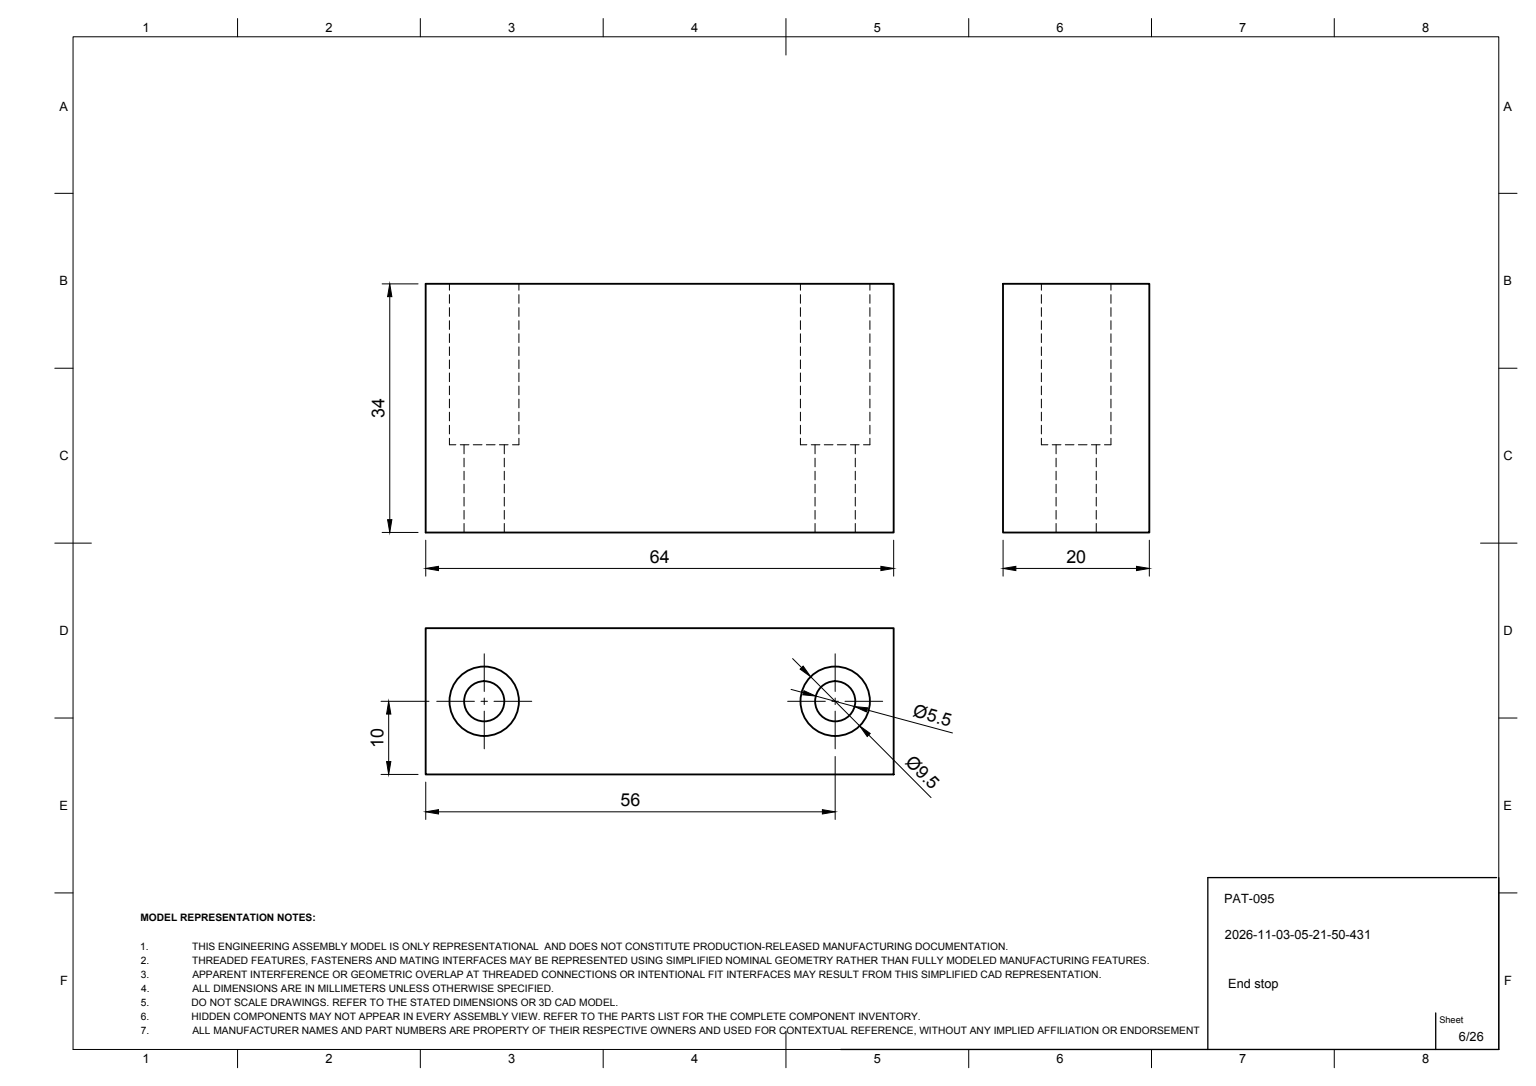
ISO-10303-21;
HEADER;
/* Generated by software containing ST-Developer
 * from STEP Tools, Inc. (www.steptools.com) 
 */

FILE_DESCRIPTION(
/* description */ ('Single-Axis Profile-Rail Linear Slide'),
/* implementation_level */ '2;1');

FILE_NAME(
/* name */ 'End stop.step',
/* time_stamp */ '2026-10-27T10:47:43-07:00',
/* author */ (''),
/* organization */ (''),
/* preprocessor_version */ 'ST-DEVELOPER v20.2',
/* originating_system */ 'Autodesk Translation Framework v15.17.0.0',
/* authorisation */ '');

FILE_SCHEMA (('AUTOMOTIVE_DESIGN { 1 0 10303 214 3 1 1 }'));
ENDSEC;

DATA;
#10=MECHANICAL_DESIGN_GEOMETRIC_PRESENTATION_REPRESENTATION('',(#330),#14478);
#276=SHAPE_REPRESENTATION_RELATIONSHIP('SRR','None',#14606,#303);
#303=ADVANCED_BREP_SHAPE_REPRESENTATION('',(#357),#14450);
#330=STYLED_ITEM('',(#14824),#357);
#357=MANIFOLD_SOLID_BREP('Body1',#8590);
#406=FACE_BOUND('',#1345,.T.);
#407=FACE_BOUND('',#1348,.T.);
#408=FACE_BOUND('',#1356,.T.);
#409=FACE_BOUND('',#1357,.T.);
#410=FACE_BOUND('',#1359,.T.);
#411=FACE_BOUND('',#1360,.T.);
#474=PLANE('',#8974);
#475=PLANE('',#8979);
#476=PLANE('',#8985);
#477=PLANE('',#8986);
#478=PLANE('',#8987);
#479=PLANE('',#8988);
#480=PLANE('',#8989);
#481=PLANE('',#8990);
#860=FACE_OUTER_BOUND('',#1343,.T.);
#861=FACE_OUTER_BOUND('',#1344,.T.);
#862=FACE_OUTER_BOUND('',#1346,.T.);
#863=FACE_OUTER_BOUND('',#1347,.T.);
#864=FACE_OUTER_BOUND('',#1349,.T.);
#865=FACE_OUTER_BOUND('',#1350,.T.);
#866=FACE_OUTER_BOUND('',#1351,.T.);
#867=FACE_OUTER_BOUND('',#1352,.T.);
#868=FACE_OUTER_BOUND('',#1353,.T.);
#869=FACE_OUTER_BOUND('',#1354,.T.);
#870=FACE_OUTER_BOUND('',#1355,.T.);
#871=FACE_OUTER_BOUND('',#1358,.T.);
#1343=EDGE_LOOP('',(#5921,#5922,#5923,#5924));
#1344=EDGE_LOOP('',(#5925));
#1345=EDGE_LOOP('',(#5926));
#1346=EDGE_LOOP('',(#5927,#5928,#5929,#5930));
#1347=EDGE_LOOP('',(#5931));
#1348=EDGE_LOOP('',(#5932));
#1349=EDGE_LOOP('',(#5933,#5934,#5935,#5936));
#1350=EDGE_LOOP('',(#5937,#5938,#5939,#5940));
#1351=EDGE_LOOP('',(#5941,#5942,#5943,#5944));
#1352=EDGE_LOOP('',(#5945,#5946,#5947,#5948));
#1353=EDGE_LOOP('',(#5949,#5950,#5951,#5952));
#1354=EDGE_LOOP('',(#5953,#5954,#5955,#5956));
#1355=EDGE_LOOP('',(#5957,#5958,#5959,#5960));
#1356=EDGE_LOOP('',(#5961));
#1357=EDGE_LOOP('',(#5962));
#1358=EDGE_LOOP('',(#5963,#5964,#5965,#5966));
#1359=EDGE_LOOP('',(#5967));
#1360=EDGE_LOOP('',(#5968));
#1866=LINE('',#12114,#2837);
#1867=LINE('',#12123,#2838);
#1868=LINE('',#12131,#2839);
#1869=LINE('',#12135,#2840);
#1870=LINE('',#12139,#2841);
#1871=LINE('',#12141,#2842);
#1872=LINE('',#12143,#2843);
#1873=LINE('',#12144,#2844);
#1874=LINE('',#12147,#2845);
#1875=LINE('',#12149,#2846);
#1876=LINE('',#12150,#2847);
#1877=LINE('',#12153,#2848);
#1878=LINE('',#12155,#2849);
#1879=LINE('',#12156,#2850);
#1880=LINE('',#12158,#2851);
#1881=LINE('',#12159,#2852);
#2837=VECTOR('',#9755,0.475);
#2838=VECTOR('',#9766,0.475);
#2839=VECTOR('',#9777,0.275);
#2840=VECTOR('',#9782,0.275);
#2841=VECTOR('',#9785,1.);
#2842=VECTOR('',#9786,1.);
#2843=VECTOR('',#9787,1.);
#2844=VECTOR('',#9788,1.);
#2845=VECTOR('',#9791,1.);
#2846=VECTOR('',#9792,1.);
#2847=VECTOR('',#9793,1.);
#2848=VECTOR('',#9796,1.);
#2849=VECTOR('',#9797,1.);
#2850=VECTOR('',#9798,1.);
#2851=VECTOR('',#9801,1.);
#2852=VECTOR('',#9802,1.);
#3810=CIRCLE('',#8972,0.475);
#3811=CIRCLE('',#8973,0.475);
#3812=CIRCLE('',#8975,0.275);
#3813=CIRCLE('',#8977,0.475);
#3814=CIRCLE('',#8978,0.475);
#3815=CIRCLE('',#8980,0.275);
#3816=CIRCLE('',#8982,0.275);
#3817=CIRCLE('',#8984,0.275);
#3974=VERTEX_POINT('',#12111);
#3975=VERTEX_POINT('',#12113);
#3976=VERTEX_POINT('',#12117);
#3977=VERTEX_POINT('',#12120);
#3978=VERTEX_POINT('',#12122);
#3979=VERTEX_POINT('',#12126);
#3980=VERTEX_POINT('',#12129);
#3981=VERTEX_POINT('',#12133);
#3982=VERTEX_POINT('',#12137);
#3983=VERTEX_POINT('',#12138);
#3984=VERTEX_POINT('',#12140);
#3985=VERTEX_POINT('',#12142);
#3986=VERTEX_POINT('',#12146);
#3987=VERTEX_POINT('',#12148);
#3988=VERTEX_POINT('',#12152);
#3989=VERTEX_POINT('',#12154);
#4738=EDGE_CURVE('',#3974,#3974,#3810,.T.);
#4739=EDGE_CURVE('',#3974,#3975,#1866,.T.);
#4740=EDGE_CURVE('',#3975,#3975,#3811,.T.);
#4741=EDGE_CURVE('',#3976,#3976,#3812,.T.);
#4742=EDGE_CURVE('',#3977,#3977,#3813,.T.);
#4743=EDGE_CURVE('',#3977,#3978,#1867,.T.);
#4744=EDGE_CURVE('',#3978,#3978,#3814,.T.);
#4745=EDGE_CURVE('',#3979,#3979,#3815,.T.);
#4746=EDGE_CURVE('',#3980,#3980,#3816,.T.);
#4747=EDGE_CURVE('',#3980,#3976,#1868,.T.);
#4748=EDGE_CURVE('',#3981,#3981,#3817,.T.);
#4749=EDGE_CURVE('',#3981,#3979,#1869,.T.);
#4750=EDGE_CURVE('',#3982,#3983,#1870,.T.);
#4751=EDGE_CURVE('',#3983,#3984,#1871,.T.);
#4752=EDGE_CURVE('',#3985,#3984,#1872,.T.);
#4753=EDGE_CURVE('',#3982,#3985,#1873,.T.);
#4754=EDGE_CURVE('',#3986,#3982,#1874,.T.);
#4755=EDGE_CURVE('',#3987,#3985,#1875,.T.);
#4756=EDGE_CURVE('',#3986,#3987,#1876,.T.);
#4757=EDGE_CURVE('',#3988,#3986,#1877,.T.);
#4758=EDGE_CURVE('',#3989,#3987,#1878,.T.);
#4759=EDGE_CURVE('',#3988,#3989,#1879,.T.);
#4760=EDGE_CURVE('',#3983,#3988,#1880,.T.);
#4761=EDGE_CURVE('',#3984,#3989,#1881,.T.);
#5921=ORIENTED_EDGE('',*,*,#4738,.F.);
#5922=ORIENTED_EDGE('',*,*,#4739,.T.);
#5923=ORIENTED_EDGE('',*,*,#4740,.F.);
#5924=ORIENTED_EDGE('',*,*,#4739,.F.);
#5925=ORIENTED_EDGE('',*,*,#4738,.T.);
#5926=ORIENTED_EDGE('',*,*,#4741,.F.);
#5927=ORIENTED_EDGE('',*,*,#4742,.F.);
#5928=ORIENTED_EDGE('',*,*,#4743,.T.);
#5929=ORIENTED_EDGE('',*,*,#4744,.F.);
#5930=ORIENTED_EDGE('',*,*,#4743,.F.);
#5931=ORIENTED_EDGE('',*,*,#4742,.T.);
#5932=ORIENTED_EDGE('',*,*,#4745,.F.);
#5933=ORIENTED_EDGE('',*,*,#4746,.F.);
#5934=ORIENTED_EDGE('',*,*,#4747,.T.);
#5935=ORIENTED_EDGE('',*,*,#4741,.T.);
#5936=ORIENTED_EDGE('',*,*,#4747,.F.);
#5937=ORIENTED_EDGE('',*,*,#4748,.F.);
#5938=ORIENTED_EDGE('',*,*,#4749,.T.);
#5939=ORIENTED_EDGE('',*,*,#4745,.T.);
#5940=ORIENTED_EDGE('',*,*,#4749,.F.);
#5941=ORIENTED_EDGE('',*,*,#4750,.T.);
#5942=ORIENTED_EDGE('',*,*,#4751,.T.);
#5943=ORIENTED_EDGE('',*,*,#4752,.F.);
#5944=ORIENTED_EDGE('',*,*,#4753,.F.);
#5945=ORIENTED_EDGE('',*,*,#4754,.T.);
#5946=ORIENTED_EDGE('',*,*,#4753,.T.);
#5947=ORIENTED_EDGE('',*,*,#4755,.F.);
#5948=ORIENTED_EDGE('',*,*,#4756,.F.);
#5949=ORIENTED_EDGE('',*,*,#4757,.T.);
#5950=ORIENTED_EDGE('',*,*,#4756,.T.);
#5951=ORIENTED_EDGE('',*,*,#4758,.F.);
#5952=ORIENTED_EDGE('',*,*,#4759,.F.);
#5953=ORIENTED_EDGE('',*,*,#4760,.T.);
#5954=ORIENTED_EDGE('',*,*,#4759,.T.);
#5955=ORIENTED_EDGE('',*,*,#4761,.F.);
#5956=ORIENTED_EDGE('',*,*,#4751,.F.);
#5957=ORIENTED_EDGE('',*,*,#4761,.T.);
#5958=ORIENTED_EDGE('',*,*,#4758,.T.);
#5959=ORIENTED_EDGE('',*,*,#4755,.T.);
#5960=ORIENTED_EDGE('',*,*,#4752,.T.);
#5961=ORIENTED_EDGE('',*,*,#4740,.T.);
#5962=ORIENTED_EDGE('',*,*,#4744,.T.);
#5963=ORIENTED_EDGE('',*,*,#4760,.F.);
#5964=ORIENTED_EDGE('',*,*,#4750,.F.);
#5965=ORIENTED_EDGE('',*,*,#4754,.F.);
#5966=ORIENTED_EDGE('',*,*,#4757,.F.);
#5967=ORIENTED_EDGE('',*,*,#4746,.T.);
#5968=ORIENTED_EDGE('',*,*,#4748,.T.);
#8085=CYLINDRICAL_SURFACE('',#8971,0.475);
#8086=CYLINDRICAL_SURFACE('',#8976,0.475);
#8087=CYLINDRICAL_SURFACE('',#8981,0.275);
#8088=CYLINDRICAL_SURFACE('',#8983,0.275);
#8154=ADVANCED_FACE('',(#860),#8085,.F.);
#8155=ADVANCED_FACE('',(#861,#406),#474,.T.);
#8156=ADVANCED_FACE('',(#862),#8086,.F.);
#8157=ADVANCED_FACE('',(#863,#407),#475,.T.);
#8158=ADVANCED_FACE('',(#864),#8087,.F.);
#8159=ADVANCED_FACE('',(#865),#8088,.F.);
#8160=ADVANCED_FACE('',(#866),#476,.T.);
#8161=ADVANCED_FACE('',(#867),#477,.T.);
#8162=ADVANCED_FACE('',(#868),#478,.T.);
#8163=ADVANCED_FACE('',(#869),#479,.T.);
#8164=ADVANCED_FACE('',(#870,#408,#409),#480,.T.);
#8165=ADVANCED_FACE('',(#871,#410,#411),#481,.F.);
#8590=CLOSED_SHELL('',(#8154,#8155,#8156,#8157,#8158,#8159,#8160,#8161,
#8162,#8163,#8164,#8165));
#8970=AXIS2_PLACEMENT_3D('',#12109,#9749,#9750);
#8971=AXIS2_PLACEMENT_3D('',#12110,#9751,#9752);
#8972=AXIS2_PLACEMENT_3D('',#12112,#9753,#9754);
#8973=AXIS2_PLACEMENT_3D('',#12115,#9756,#9757);
#8974=AXIS2_PLACEMENT_3D('',#12116,#9758,#9759);
#8975=AXIS2_PLACEMENT_3D('',#12118,#9760,#9761);
#8976=AXIS2_PLACEMENT_3D('',#12119,#9762,#9763);
#8977=AXIS2_PLACEMENT_3D('',#12121,#9764,#9765);
#8978=AXIS2_PLACEMENT_3D('',#12124,#9767,#9768);
#8979=AXIS2_PLACEMENT_3D('',#12125,#9769,#9770);
#8980=AXIS2_PLACEMENT_3D('',#12127,#9771,#9772);
#8981=AXIS2_PLACEMENT_3D('',#12128,#9773,#9774);
#8982=AXIS2_PLACEMENT_3D('',#12130,#9775,#9776);
#8983=AXIS2_PLACEMENT_3D('',#12132,#9778,#9779);
#8984=AXIS2_PLACEMENT_3D('',#12134,#9780,#9781);
#8985=AXIS2_PLACEMENT_3D('',#12136,#9783,#9784);
#8986=AXIS2_PLACEMENT_3D('',#12145,#9789,#9790);
#8987=AXIS2_PLACEMENT_3D('',#12151,#9794,#9795);
#8988=AXIS2_PLACEMENT_3D('',#12157,#9799,#9800);
#8989=AXIS2_PLACEMENT_3D('',#12160,#9803,#9804);
#8990=AXIS2_PLACEMENT_3D('',#12161,#9805,#9806);
#9749=DIRECTION('axis',(0.,0.,1.));
#9750=DIRECTION('refdir',(1.,0.,0.));
#9751=DIRECTION('center_axis',(0.,0.,1.));
#9752=DIRECTION('ref_axis',(1.,0.,0.));
#9753=DIRECTION('center_axis',(0.,0.,1.));
#9754=DIRECTION('ref_axis',(1.,0.,0.));
#9755=DIRECTION('',(0.,0.,1.));
#9756=DIRECTION('center_axis',(0.,0.,-1.));
#9757=DIRECTION('ref_axis',(1.,0.,0.));
#9758=DIRECTION('center_axis',(0.,0.,1.));
#9759=DIRECTION('ref_axis',(1.,0.,0.));
#9760=DIRECTION('center_axis',(0.,0.,1.));
#9761=DIRECTION('ref_axis',(1.,0.,0.));
#9762=DIRECTION('center_axis',(0.,0.,1.));
#9763=DIRECTION('ref_axis',(1.,0.,0.));
#9764=DIRECTION('center_axis',(0.,0.,1.));
#9765=DIRECTION('ref_axis',(1.,0.,0.));
#9766=DIRECTION('',(0.,0.,1.));
#9767=DIRECTION('center_axis',(0.,0.,-1.));
#9768=DIRECTION('ref_axis',(1.,0.,0.));
#9769=DIRECTION('center_axis',(0.,0.,1.));
#9770=DIRECTION('ref_axis',(1.,0.,0.));
#9771=DIRECTION('center_axis',(0.,0.,1.));
#9772=DIRECTION('ref_axis',(1.,0.,0.));
#9773=DIRECTION('center_axis',(0.,0.,1.));
#9774=DIRECTION('ref_axis',(1.,0.,0.));
#9775=DIRECTION('center_axis',(0.,0.,1.));
#9776=DIRECTION('ref_axis',(1.,0.,0.));
#9777=DIRECTION('',(0.,0.,1.));
#9778=DIRECTION('center_axis',(0.,0.,1.));
#9779=DIRECTION('ref_axis',(1.,0.,0.));
#9780=DIRECTION('center_axis',(0.,0.,1.));
#9781=DIRECTION('ref_axis',(1.,0.,0.));
#9782=DIRECTION('',(0.,0.,1.));
#9783=DIRECTION('center_axis',(0.,1.,0.));
#9784=DIRECTION('ref_axis',(-1.,0.,0.));
#9785=DIRECTION('',(-1.,0.,0.));
#9786=DIRECTION('',(0.,0.,1.));
#9787=DIRECTION('',(-1.,0.,0.));
#9788=DIRECTION('',(0.,0.,1.));
#9789=DIRECTION('center_axis',(1.,0.,0.));
#9790=DIRECTION('ref_axis',(0.,1.,0.));
#9791=DIRECTION('',(0.,1.,0.));
#9792=DIRECTION('',(0.,1.,0.));
#9793=DIRECTION('',(0.,0.,1.));
#9794=DIRECTION('center_axis',(0.,-1.,0.));
#9795=DIRECTION('ref_axis',(1.,0.,0.));
#9796=DIRECTION('',(1.,0.,0.));
#9797=DIRECTION('',(1.,0.,0.));
#9798=DIRECTION('',(0.,0.,1.));
#9799=DIRECTION('center_axis',(-1.,0.,0.));
#9800=DIRECTION('ref_axis',(0.,-1.,0.));
#9801=DIRECTION('',(0.,-1.,0.));
#9802=DIRECTION('',(0.,-1.,0.));
#9803=DIRECTION('center_axis',(0.,0.,1.));
#9804=DIRECTION('ref_axis',(1.,0.,0.));
#9805=DIRECTION('center_axis',(0.,0.,1.));
#9806=DIRECTION('ref_axis',(1.,0.,0.));
#12109=CARTESIAN_POINT('',(0.,0.,0.));
#12110=CARTESIAN_POINT('Origin',(-1.,-2.4,4.));
#12111=CARTESIAN_POINT('',(-1.475,-2.4,4.));
#12112=CARTESIAN_POINT('Origin',(-1.,-2.4,4.));
#12113=CARTESIAN_POINT('',(-1.475,-2.4,6.2));
#12114=CARTESIAN_POINT('',(-1.475,-2.4,4.));
#12115=CARTESIAN_POINT('Origin',(-1.,-2.4,6.2));
#12116=CARTESIAN_POINT('Origin',(-1.,-2.4,4.));
#12117=CARTESIAN_POINT('',(-1.275,-2.4,4.));
#12118=CARTESIAN_POINT('Origin',(-1.,-2.4,4.));
#12119=CARTESIAN_POINT('Origin',(-1.,2.4,4.));
#12120=CARTESIAN_POINT('',(-1.475,2.4,4.));
#12121=CARTESIAN_POINT('Origin',(-1.,2.4,4.));
#12122=CARTESIAN_POINT('',(-1.475,2.4,6.2));
#12123=CARTESIAN_POINT('',(-1.475,2.4,4.));
#12124=CARTESIAN_POINT('Origin',(-1.,2.4,6.2));
#12125=CARTESIAN_POINT('Origin',(-1.,2.4,4.));
#12126=CARTESIAN_POINT('',(-1.275,2.4,4.));
#12127=CARTESIAN_POINT('Origin',(-1.,2.4,4.));
#12128=CARTESIAN_POINT('Origin',(-1.,-2.4,2.7));
#12129=CARTESIAN_POINT('',(-1.275,-2.4,2.8));
#12130=CARTESIAN_POINT('Origin',(-1.,-2.4,2.8));
#12131=CARTESIAN_POINT('',(-1.275,-2.4,2.7));
#12132=CARTESIAN_POINT('Origin',(-1.,2.4,2.7));
#12133=CARTESIAN_POINT('',(-1.275,2.4,2.8));
#12134=CARTESIAN_POINT('Origin',(-1.,2.4,2.8));
#12135=CARTESIAN_POINT('',(-1.275,2.4,2.7));
#12136=CARTESIAN_POINT('Origin',(0.,3.2,2.8));
#12137=CARTESIAN_POINT('',(0.,3.2,2.8));
#12138=CARTESIAN_POINT('',(-2.,3.2,2.8));
#12139=CARTESIAN_POINT('',(0.,3.2,2.8));
#12140=CARTESIAN_POINT('',(-2.,3.2,6.2));
#12141=CARTESIAN_POINT('',(-2.,3.2,2.8));
#12142=CARTESIAN_POINT('',(0.,3.2,6.2));
#12143=CARTESIAN_POINT('',(0.,3.2,6.2));
#12144=CARTESIAN_POINT('',(0.,3.2,2.8));
#12145=CARTESIAN_POINT('Origin',(0.,-3.2,2.8));
#12146=CARTESIAN_POINT('',(0.,-3.2,2.8));
#12147=CARTESIAN_POINT('',(0.,-3.2,2.8));
#12148=CARTESIAN_POINT('',(0.,-3.2,6.2));
#12149=CARTESIAN_POINT('',(0.,-3.2,6.2));
#12150=CARTESIAN_POINT('',(0.,-3.2,2.8));
#12151=CARTESIAN_POINT('Origin',(-2.,-3.2,2.8));
#12152=CARTESIAN_POINT('',(-2.,-3.2,2.8));
#12153=CARTESIAN_POINT('',(-2.,-3.2,2.8));
#12154=CARTESIAN_POINT('',(-2.,-3.2,6.2));
#12155=CARTESIAN_POINT('',(-2.,-3.2,6.2));
#12156=CARTESIAN_POINT('',(-2.,-3.2,2.8));
#12157=CARTESIAN_POINT('Origin',(-2.,3.2,2.8));
#12158=CARTESIAN_POINT('',(-2.,3.2,2.8));
#12159=CARTESIAN_POINT('',(-2.,3.2,6.2));
#12160=CARTESIAN_POINT('Origin',(-1.,0.,6.2));
#12161=CARTESIAN_POINT('Origin',(-1.,0.,2.8));
#14418=UNCERTAINTY_MEASURE_WITH_UNIT(LENGTH_MEASURE(0.001),#14479,
'DISTANCE_ACCURACY_VALUE',
'Maximum model space distance between geometric entities at asserted c
onnectivities');
#14446=UNCERTAINTY_MEASURE_WITH_UNIT(LENGTH_MEASURE(0.001),#14479,
'DISTANCE_ACCURACY_VALUE',
'Maximum model space distance between geometric entities at asserted c
onnectivities');
#14450=(
GEOMETRIC_REPRESENTATION_CONTEXT(3)
GLOBAL_UNCERTAINTY_ASSIGNED_CONTEXT((#14418))
GLOBAL_UNIT_ASSIGNED_CONTEXT((#14479,#14481,#14482))
REPRESENTATION_CONTEXT('','3D')
);
#14478=(
GEOMETRIC_REPRESENTATION_CONTEXT(3)
GLOBAL_UNCERTAINTY_ASSIGNED_CONTEXT((#14446))
GLOBAL_UNIT_ASSIGNED_CONTEXT((#14479,#14481,#14482))
REPRESENTATION_CONTEXT('','3D')
);
#14479=(
LENGTH_UNIT()
NAMED_UNIT(*)
SI_UNIT(.CENTI.,.METRE.)
);
#14481=(
NAMED_UNIT(*)
PLANE_ANGLE_UNIT()
SI_UNIT($,.RADIAN.)
);
#14482=(
NAMED_UNIT(*)
SI_UNIT($,.STERADIAN.)
SOLID_ANGLE_UNIT()
);
#14486=SHAPE_DEFINITION_REPRESENTATION(#14517,#14606);
#14517=PRODUCT_DEFINITION_SHAPE('',$,#14638);
#14606=SHAPE_REPRESENTATION('',(#8970),#14450);
#14634=PRODUCT_DEFINITION_CONTEXT('part definition',#14729,'design');
#14638=PRODUCT_DEFINITION('End stop','End stop',#14669,#14634);
#14669=PRODUCT_DEFINITION_FORMATION('',$,#14734);
#14729=APPLICATION_CONTEXT(
'Core Data for Automotive Mechanical Design Process');
#14730=PRODUCT_CONTEXT('part definition',#14729,'mechanical');
#14734=PRODUCT('End stop','End stop','End stop',(#14730));
#14818=COLOUR_RGB('Sky Blue',0.24,0.69,0.87);
#14819=FILL_AREA_STYLE_COLOUR('',#14818);
#14820=FILL_AREA_STYLE('',(#14819));
#14821=SURFACE_STYLE_FILL_AREA(#14820);
#14822=SURFACE_SIDE_STYLE('',(#14821));
#14823=SURFACE_STYLE_USAGE(.BOTH.,#14822);
#14824=PRESENTATION_STYLE_ASSIGNMENT((#14823));
ENDSEC;
END-ISO-10303-21;
